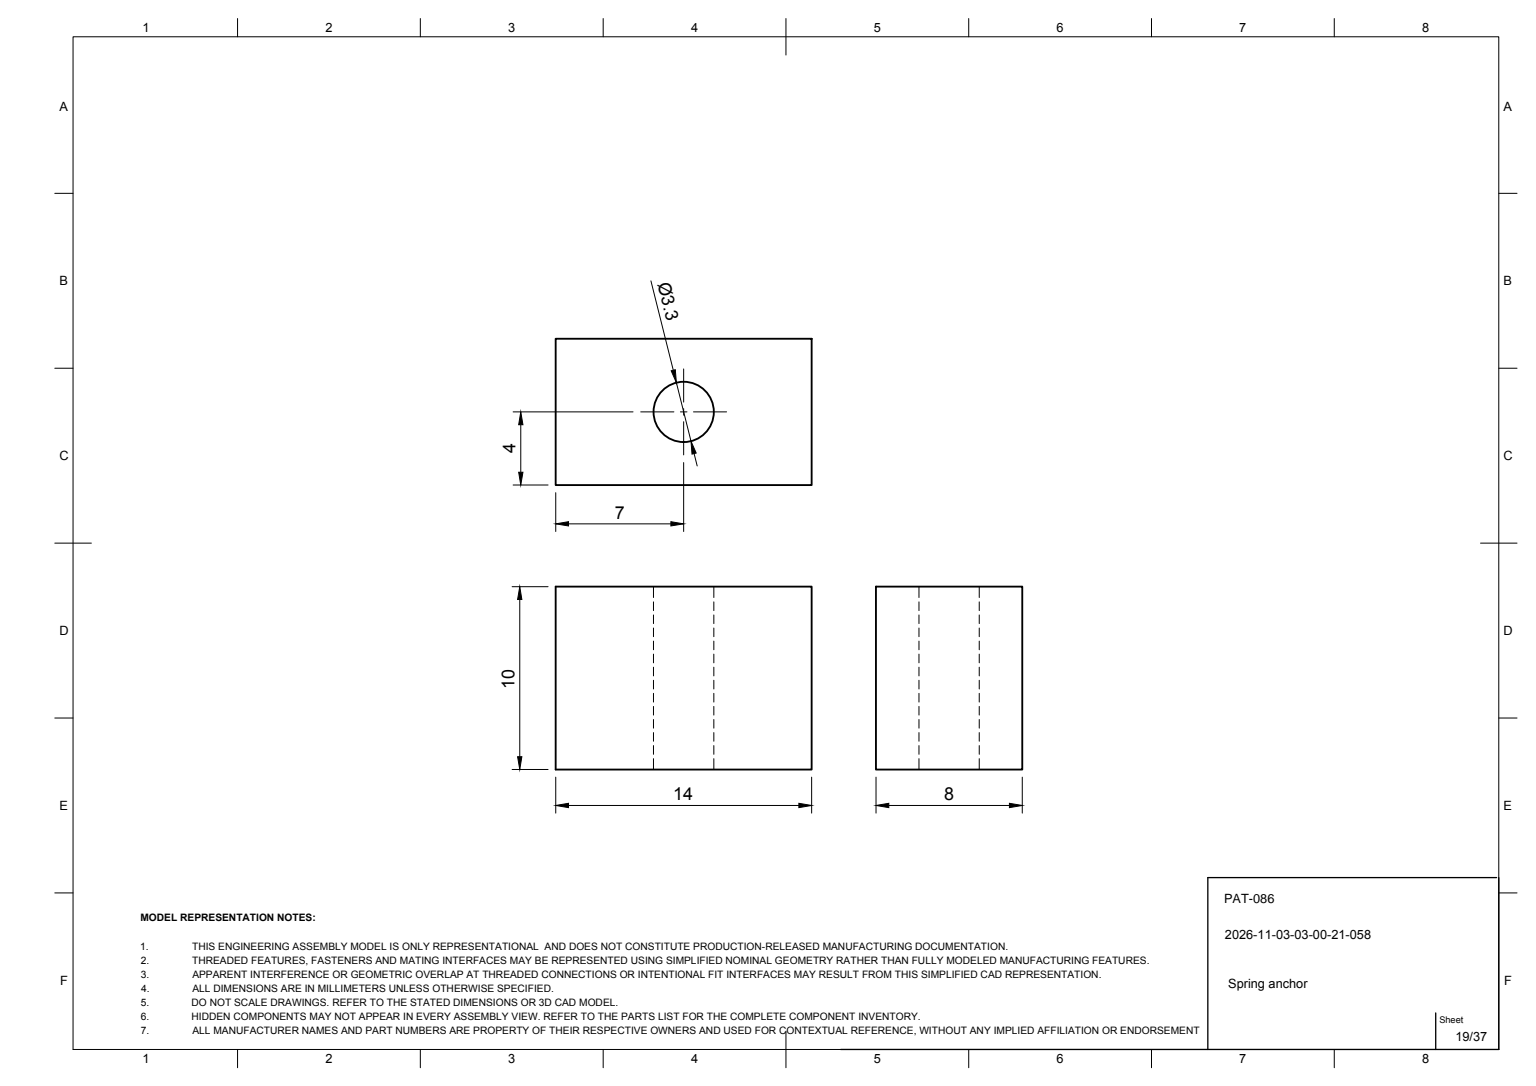
ISO-10303-21;
HEADER;
/* Generated by software containing ST-Developer
 * from STEP Tools, Inc. (www.steptools.com) 
 */

FILE_DESCRIPTION(
/* description */ ('Ratchet and pawl hand winch drum'),
/* implementation_level */ '2;1');

FILE_NAME(
/* name */ 'Spring anchor.step',
/* time_stamp */ '2026-10-27T12:42:58-07:00',
/* author */ (''),
/* organization */ (''),
/* preprocessor_version */ 'ST-DEVELOPER v20.2',
/* originating_system */ 'Autodesk Translation Framework v15.17.0.0',
/* authorisation */ '');

FILE_SCHEMA (('AUTOMOTIVE_DESIGN { 1 0 10303 214 3 1 1 }'));
ENDSEC;

DATA;
#10=MECHANICAL_DESIGN_GEOMETRIC_PRESENTATION_REPRESENTATION('',(#403),#11801);
#335=SHAPE_REPRESENTATION_RELATIONSHIP('SRR','None',#11961,#369);
#369=ADVANCED_BREP_SHAPE_REPRESENTATION('',(#438),#11778);
#403=STYLED_ITEM('',(#12213),#438);
#438=MANIFOLD_SOLID_BREP('Body1',#6280);
#529=FACE_BOUND('',#1394,.T.);
#530=FACE_BOUND('',#1396,.T.);
#672=PLANE('',#6914);
#673=PLANE('',#6915);
#674=PLANE('',#6916);
#675=PLANE('',#6917);
#676=PLANE('',#6918);
#677=PLANE('',#6919);
#959=FACE_OUTER_BOUND('',#1388,.T.);
#960=FACE_OUTER_BOUND('',#1389,.T.);
#961=FACE_OUTER_BOUND('',#1390,.T.);
#962=FACE_OUTER_BOUND('',#1391,.T.);
#963=FACE_OUTER_BOUND('',#1392,.T.);
#964=FACE_OUTER_BOUND('',#1393,.T.);
#965=FACE_OUTER_BOUND('',#1395,.T.);
#1388=EDGE_LOOP('',(#4727,#4728,#4729,#4730));
#1389=EDGE_LOOP('',(#4731,#4732,#4733,#4734));
#1390=EDGE_LOOP('',(#4735,#4736,#4737,#4738));
#1391=EDGE_LOOP('',(#4739,#4740,#4741,#4742));
#1392=EDGE_LOOP('',(#4743,#4744,#4745,#4746));
#1393=EDGE_LOOP('',(#4747,#4748,#4749,#4750));
#1394=EDGE_LOOP('',(#4751));
#1395=EDGE_LOOP('',(#4752,#4753,#4754,#4755));
#1396=EDGE_LOOP('',(#4756));
#1841=LINE('',#9767,#2352);
#1842=LINE('',#9772,#2353);
#1843=LINE('',#9774,#2354);
#1844=LINE('',#9776,#2355);
#1845=LINE('',#9777,#2356);
#1846=LINE('',#9780,#2357);
#1847=LINE('',#9782,#2358);
#1848=LINE('',#9783,#2359);
#1849=LINE('',#9786,#2360);
#1850=LINE('',#9788,#2361);
#1851=LINE('',#9789,#2362);
#1852=LINE('',#9791,#2363);
#1853=LINE('',#9792,#2364);
#2352=VECTOR('',#7970,0.164999999999999);
#2353=VECTOR('',#7975,1.);
#2354=VECTOR('',#7976,1.);
#2355=VECTOR('',#7977,1.);
#2356=VECTOR('',#7978,1.);
#2357=VECTOR('',#7981,1.);
#2358=VECTOR('',#7982,1.);
#2359=VECTOR('',#7983,1.);
#2360=VECTOR('',#7986,1.);
#2361=VECTOR('',#7987,1.);
#2362=VECTOR('',#7988,1.);
#2363=VECTOR('',#7991,1.);
#2364=VECTOR('',#7992,1.);
#2815=CIRCLE('',#6912,0.164999999999999);
#2816=CIRCLE('',#6913,0.164999999999999);
#3102=VERTEX_POINT('',#9764);
#3103=VERTEX_POINT('',#9766);
#3104=VERTEX_POINT('',#9770);
#3105=VERTEX_POINT('',#9771);
#3106=VERTEX_POINT('',#9773);
#3107=VERTEX_POINT('',#9775);
#3108=VERTEX_POINT('',#9779);
#3109=VERTEX_POINT('',#9781);
#3110=VERTEX_POINT('',#9785);
#3111=VERTEX_POINT('',#9787);
#3707=EDGE_CURVE('',#3102,#3102,#2815,.T.);
#3708=EDGE_CURVE('',#3102,#3103,#1841,.T.);
#3709=EDGE_CURVE('',#3103,#3103,#2816,.T.);
#3710=EDGE_CURVE('',#3104,#3105,#1842,.T.);
#3711=EDGE_CURVE('',#3105,#3106,#1843,.T.);
#3712=EDGE_CURVE('',#3107,#3106,#1844,.T.);
#3713=EDGE_CURVE('',#3104,#3107,#1845,.T.);
#3714=EDGE_CURVE('',#3108,#3104,#1846,.T.);
#3715=EDGE_CURVE('',#3109,#3107,#1847,.T.);
#3716=EDGE_CURVE('',#3108,#3109,#1848,.T.);
#3717=EDGE_CURVE('',#3110,#3108,#1849,.T.);
#3718=EDGE_CURVE('',#3111,#3109,#1850,.T.);
#3719=EDGE_CURVE('',#3110,#3111,#1851,.T.);
#3720=EDGE_CURVE('',#3105,#3110,#1852,.T.);
#3721=EDGE_CURVE('',#3106,#3111,#1853,.T.);
#4727=ORIENTED_EDGE('',*,*,#3707,.F.);
#4728=ORIENTED_EDGE('',*,*,#3708,.T.);
#4729=ORIENTED_EDGE('',*,*,#3709,.F.);
#4730=ORIENTED_EDGE('',*,*,#3708,.F.);
#4731=ORIENTED_EDGE('',*,*,#3710,.T.);
#4732=ORIENTED_EDGE('',*,*,#3711,.T.);
#4733=ORIENTED_EDGE('',*,*,#3712,.F.);
#4734=ORIENTED_EDGE('',*,*,#3713,.F.);
#4735=ORIENTED_EDGE('',*,*,#3714,.T.);
#4736=ORIENTED_EDGE('',*,*,#3713,.T.);
#4737=ORIENTED_EDGE('',*,*,#3715,.F.);
#4738=ORIENTED_EDGE('',*,*,#3716,.F.);
#4739=ORIENTED_EDGE('',*,*,#3717,.T.);
#4740=ORIENTED_EDGE('',*,*,#3716,.T.);
#4741=ORIENTED_EDGE('',*,*,#3718,.F.);
#4742=ORIENTED_EDGE('',*,*,#3719,.F.);
#4743=ORIENTED_EDGE('',*,*,#3720,.T.);
#4744=ORIENTED_EDGE('',*,*,#3719,.T.);
#4745=ORIENTED_EDGE('',*,*,#3721,.F.);
#4746=ORIENTED_EDGE('',*,*,#3711,.F.);
#4747=ORIENTED_EDGE('',*,*,#3721,.T.);
#4748=ORIENTED_EDGE('',*,*,#3718,.T.);
#4749=ORIENTED_EDGE('',*,*,#3715,.T.);
#4750=ORIENTED_EDGE('',*,*,#3712,.T.);
#4751=ORIENTED_EDGE('',*,*,#3709,.T.);
#4752=ORIENTED_EDGE('',*,*,#3720,.F.);
#4753=ORIENTED_EDGE('',*,*,#3710,.F.);
#4754=ORIENTED_EDGE('',*,*,#3714,.F.);
#4755=ORIENTED_EDGE('',*,*,#3717,.F.);
#4756=ORIENTED_EDGE('',*,*,#3707,.T.);
#5855=CYLINDRICAL_SURFACE('',#6911,0.164999999999999);
#6029=ADVANCED_FACE('',(#959),#5855,.F.);
#6030=ADVANCED_FACE('',(#960),#672,.T.);
#6031=ADVANCED_FACE('',(#961),#673,.T.);
#6032=ADVANCED_FACE('',(#962),#674,.T.);
#6033=ADVANCED_FACE('',(#963),#675,.T.);
#6034=ADVANCED_FACE('',(#964,#529),#676,.T.);
#6035=ADVANCED_FACE('',(#965,#530),#677,.F.);
#6280=CLOSED_SHELL('',(#6029,#6030,#6031,#6032,#6033,#6034,#6035));
#6910=AXIS2_PLACEMENT_3D('',#9762,#7964,#7965);
#6911=AXIS2_PLACEMENT_3D('',#9763,#7966,#7967);
#6912=AXIS2_PLACEMENT_3D('',#9765,#7968,#7969);
#6913=AXIS2_PLACEMENT_3D('',#9768,#7971,#7972);
#6914=AXIS2_PLACEMENT_3D('',#9769,#7973,#7974);
#6915=AXIS2_PLACEMENT_3D('',#9778,#7979,#7980);
#6916=AXIS2_PLACEMENT_3D('',#9784,#7984,#7985);
#6917=AXIS2_PLACEMENT_3D('',#9790,#7989,#7990);
#6918=AXIS2_PLACEMENT_3D('',#9793,#7993,#7994);
#6919=AXIS2_PLACEMENT_3D('',#9794,#7995,#7996);
#7964=DIRECTION('axis',(0.,0.,1.));
#7965=DIRECTION('refdir',(1.,0.,0.));
#7966=DIRECTION('center_axis',(0.,0.,1.));
#7967=DIRECTION('ref_axis',(1.,0.,0.));
#7968=DIRECTION('center_axis',(0.,0.,1.));
#7969=DIRECTION('ref_axis',(1.,0.,0.));
#7970=DIRECTION('',(0.,0.,1.));
#7971=DIRECTION('center_axis',(0.,0.,-1.));
#7972=DIRECTION('ref_axis',(1.,0.,0.));
#7973=DIRECTION('center_axis',(0.,1.,0.));
#7974=DIRECTION('ref_axis',(-1.,0.,0.));
#7975=DIRECTION('',(-1.,0.,0.));
#7976=DIRECTION('',(0.,0.,1.));
#7977=DIRECTION('',(-1.,0.,0.));
#7978=DIRECTION('',(0.,0.,1.));
#7979=DIRECTION('center_axis',(1.,0.,0.));
#7980=DIRECTION('ref_axis',(0.,1.,0.));
#7981=DIRECTION('',(0.,1.,0.));
#7982=DIRECTION('',(0.,1.,0.));
#7983=DIRECTION('',(0.,0.,1.));
#7984=DIRECTION('center_axis',(0.,-1.,0.));
#7985=DIRECTION('ref_axis',(1.,0.,0.));
#7986=DIRECTION('',(1.,0.,0.));
#7987=DIRECTION('',(1.,0.,0.));
#7988=DIRECTION('',(0.,0.,1.));
#7989=DIRECTION('center_axis',(-1.,0.,0.));
#7990=DIRECTION('ref_axis',(0.,-1.,0.));
#7991=DIRECTION('',(0.,-1.,0.));
#7992=DIRECTION('',(0.,-1.,0.));
#7993=DIRECTION('center_axis',(0.,0.,1.));
#7994=DIRECTION('ref_axis',(1.,0.,0.));
#7995=DIRECTION('center_axis',(0.,0.,1.));
#7996=DIRECTION('ref_axis',(1.,0.,0.));
#9762=CARTESIAN_POINT('',(0.,0.,0.));
#9763=CARTESIAN_POINT('Origin',(8.3,-3.7,5.4));
#9764=CARTESIAN_POINT('',(8.135,-3.7,5.5));
#9765=CARTESIAN_POINT('Origin',(8.3,-3.7,5.5));
#9766=CARTESIAN_POINT('',(8.135,-3.7,6.5));
#9767=CARTESIAN_POINT('',(8.135,-3.7,5.4));
#9768=CARTESIAN_POINT('Origin',(8.3,-3.7,6.5));
#9769=CARTESIAN_POINT('Origin',(8.7,-3.,5.5));
#9770=CARTESIAN_POINT('',(8.7,-3.,5.5));
#9771=CARTESIAN_POINT('',(7.9,-3.,5.5));
#9772=CARTESIAN_POINT('',(8.7,-3.,5.5));
#9773=CARTESIAN_POINT('',(7.9,-3.,6.5));
#9774=CARTESIAN_POINT('',(7.9,-3.,5.5));
#9775=CARTESIAN_POINT('',(8.7,-3.,6.5));
#9776=CARTESIAN_POINT('',(8.7,-3.,6.5));
#9777=CARTESIAN_POINT('',(8.7,-3.,5.5));
#9778=CARTESIAN_POINT('Origin',(8.7,-4.4,5.5));
#9779=CARTESIAN_POINT('',(8.7,-4.4,5.5));
#9780=CARTESIAN_POINT('',(8.7,-4.4,5.5));
#9781=CARTESIAN_POINT('',(8.7,-4.4,6.5));
#9782=CARTESIAN_POINT('',(8.7,-4.4,6.5));
#9783=CARTESIAN_POINT('',(8.7,-4.4,5.5));
#9784=CARTESIAN_POINT('Origin',(7.9,-4.4,5.5));
#9785=CARTESIAN_POINT('',(7.9,-4.4,5.5));
#9786=CARTESIAN_POINT('',(7.9,-4.4,5.5));
#9787=CARTESIAN_POINT('',(7.9,-4.4,6.5));
#9788=CARTESIAN_POINT('',(7.9,-4.4,6.5));
#9789=CARTESIAN_POINT('',(7.9,-4.4,5.5));
#9790=CARTESIAN_POINT('Origin',(7.9,-3.,5.5));
#9791=CARTESIAN_POINT('',(7.9,-3.,5.5));
#9792=CARTESIAN_POINT('',(7.9,-3.,6.5));
#9793=CARTESIAN_POINT('Origin',(8.3,-3.7,6.5));
#9794=CARTESIAN_POINT('Origin',(8.3,-3.7,5.5));
#11738=UNCERTAINTY_MEASURE_WITH_UNIT(LENGTH_MEASURE(0.001),#11802,
'DISTANCE_ACCURACY_VALUE',
'Maximum model space distance between geometric entities at asserted c
onnectivities');
#11761=UNCERTAINTY_MEASURE_WITH_UNIT(LENGTH_MEASURE(0.001),#11802,
'DISTANCE_ACCURACY_VALUE',
'Maximum model space distance between geometric entities at asserted c
onnectivities');
#11778=(
GEOMETRIC_REPRESENTATION_CONTEXT(3)
GLOBAL_UNCERTAINTY_ASSIGNED_CONTEXT((#11738))
GLOBAL_UNIT_ASSIGNED_CONTEXT((#11802,#11804,#11805))
REPRESENTATION_CONTEXT('','3D')
);
#11801=(
GEOMETRIC_REPRESENTATION_CONTEXT(3)
GLOBAL_UNCERTAINTY_ASSIGNED_CONTEXT((#11761))
GLOBAL_UNIT_ASSIGNED_CONTEXT((#11802,#11804,#11805))
REPRESENTATION_CONTEXT('','3D')
);
#11802=(
LENGTH_UNIT()
NAMED_UNIT(*)
SI_UNIT(.CENTI.,.METRE.)
);
#11804=(
NAMED_UNIT(*)
PLANE_ANGLE_UNIT()
SI_UNIT($,.RADIAN.)
);
#11805=(
NAMED_UNIT(*)
SI_UNIT($,.STERADIAN.)
SOLID_ANGLE_UNIT()
);
#11822=SHAPE_DEFINITION_REPRESENTATION(#11861,#11961);
#11861=PRODUCT_DEFINITION_SHAPE('',$,#12001);
#11961=SHAPE_REPRESENTATION('',(#6910),#11778);
#11984=PRODUCT_DEFINITION_CONTEXT('part definition',#12103,'design');
#12001=PRODUCT_DEFINITION('Spring anchor','Spring anchor',#12040,#11984);
#12040=PRODUCT_DEFINITION_FORMATION('',$,#12121);
#12103=APPLICATION_CONTEXT(
'Core Data for Automotive Mechanical Design Process');
#12104=PRODUCT_CONTEXT('part definition',#12103,'mechanical');
#12121=PRODUCT('Spring anchor','Spring anchor','Spring anchor',(#12104));
#12207=COLOUR_RGB('Grey',0.48,0.52,0.57);
#12208=FILL_AREA_STYLE_COLOUR('',#12207);
#12209=FILL_AREA_STYLE('',(#12208));
#12210=SURFACE_STYLE_FILL_AREA(#12209);
#12211=SURFACE_SIDE_STYLE('',(#12210));
#12212=SURFACE_STYLE_USAGE(.BOTH.,#12211);
#12213=PRESENTATION_STYLE_ASSIGNMENT((#12212));
ENDSEC;
END-ISO-10303-21;
